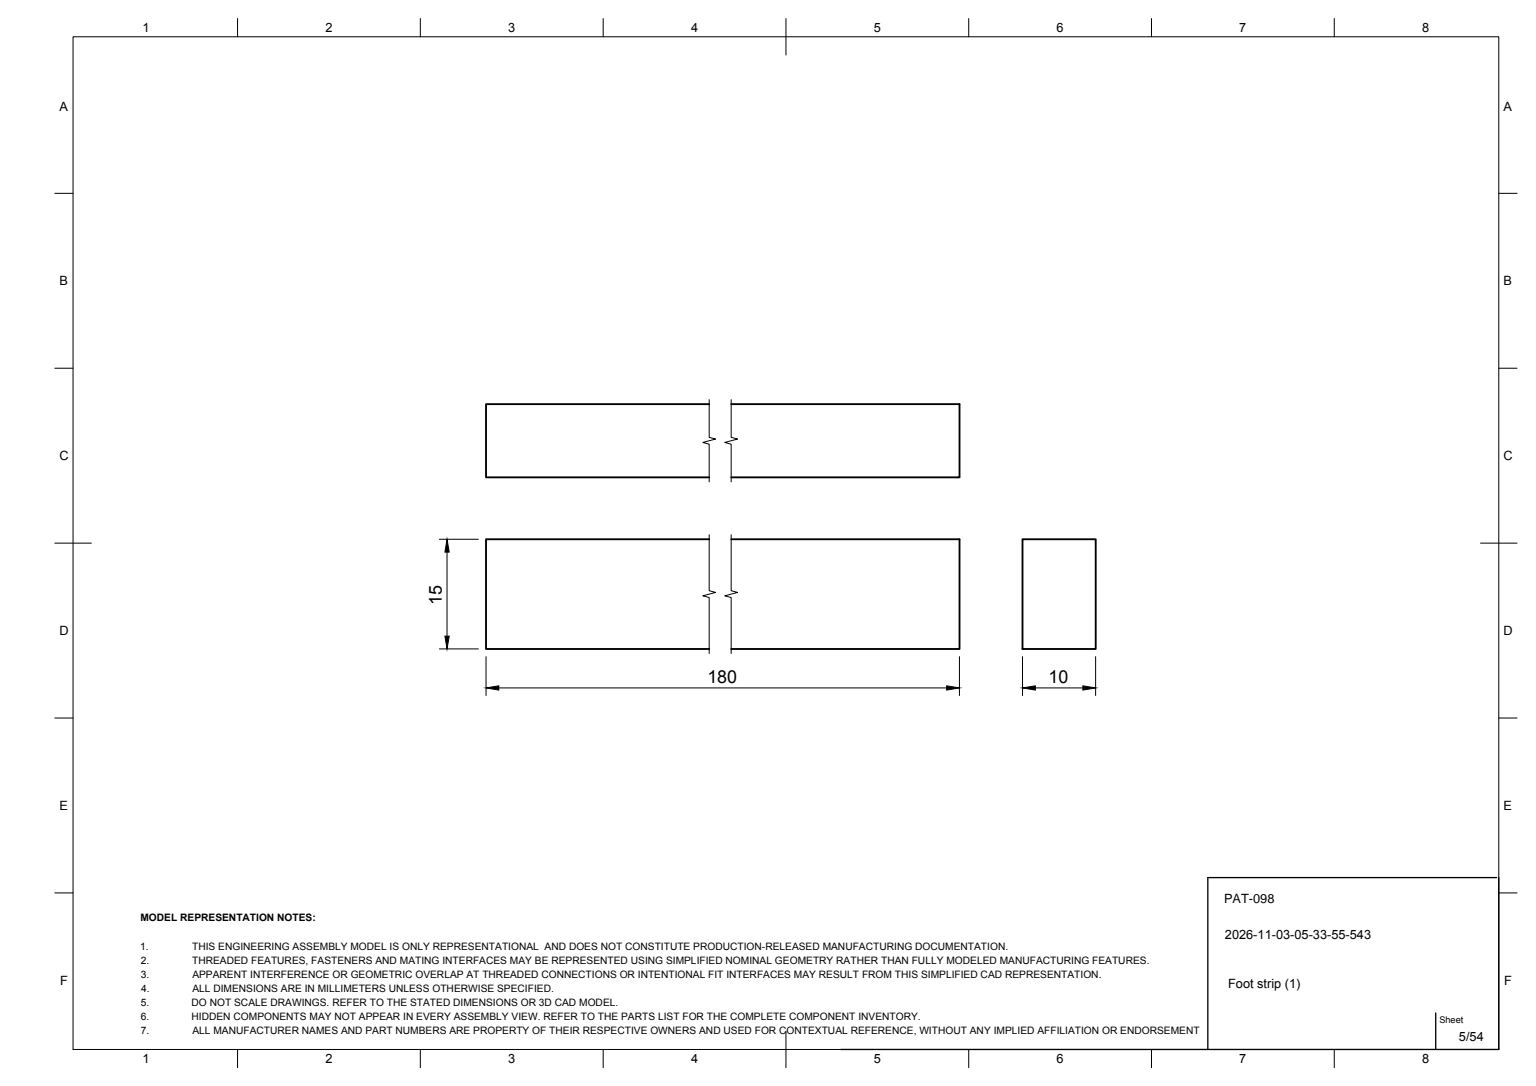
ISO-10303-21;
HEADER;
/* Generated by software containing ST-Developer
 * from STEP Tools, Inc. (www.steptools.com) 
 */

FILE_DESCRIPTION(
/* description */ ('Spring compression tester'),
/* implementation_level */ '2;1');

FILE_NAME(
/* name */ 'Foot strip (1).step',
/* time_stamp */ '2026-10-28T03:24:11-07:00',
/* author */ (''),
/* organization */ (''),
/* preprocessor_version */ 'ST-DEVELOPER v20.2',
/* originating_system */ 'Autodesk Translation Framework v15.17.0.0',
/* authorisation */ '');

FILE_SCHEMA (('AUTOMOTIVE_DESIGN { 1 0 10303 214 3 1 1 }'));
ENDSEC;

DATA;
#10=MECHANICAL_DESIGN_GEOMETRIC_PRESENTATION_REPRESENTATION('',(#1106),#43521);
#986=SHAPE_REPRESENTATION_RELATIONSHIP('SRR','None',#43798,#1046);
#1046=ADVANCED_BREP_SHAPE_REPRESENTATION('',(#1181),#43458);
#1106=STYLED_ITEM('',(#44188),#1181);
#1181=MANIFOLD_SOLID_BREP('Body1',#18543);
#1609=PLANE('',#19369);
#1610=PLANE('',#19370);
#1611=PLANE('',#19371);
#1612=PLANE('',#19372);
#1613=PLANE('',#19373);
#1614=PLANE('',#19374);
#2210=FACE_OUTER_BOUND('',#3293,.T.);
#2211=FACE_OUTER_BOUND('',#3294,.T.);
#2212=FACE_OUTER_BOUND('',#3295,.T.);
#2213=FACE_OUTER_BOUND('',#3296,.T.);
#2214=FACE_OUTER_BOUND('',#3297,.T.);
#2215=FACE_OUTER_BOUND('',#3298,.T.);
#3293=EDGE_LOOP('',(#12409,#12410,#12411,#12412));
#3294=EDGE_LOOP('',(#12413,#12414,#12415,#12416));
#3295=EDGE_LOOP('',(#12417,#12418,#12419,#12420));
#3296=EDGE_LOOP('',(#12421,#12422,#12423,#12424));
#3297=EDGE_LOOP('',(#12425,#12426,#12427,#12428));
#3298=EDGE_LOOP('',(#12429,#12430,#12431,#12432));
#4662=LINE('',#26660,#6094);
#4663=LINE('',#26662,#6095);
#4664=LINE('',#26664,#6096);
#4665=LINE('',#26665,#6097);
#4666=LINE('',#26668,#6098);
#4667=LINE('',#26670,#6099);
#4668=LINE('',#26671,#6100);
#4669=LINE('',#26674,#6101);
#4670=LINE('',#26676,#6102);
#4671=LINE('',#26677,#6103);
#4672=LINE('',#26679,#6104);
#4673=LINE('',#26680,#6105);
#6094=VECTOR('',#21424,1.);
#6095=VECTOR('',#21425,1.);
#6096=VECTOR('',#21426,1.);
#6097=VECTOR('',#21427,1.);
#6098=VECTOR('',#21430,1.);
#6099=VECTOR('',#21431,1.);
#6100=VECTOR('',#21432,1.);
#6101=VECTOR('',#21435,1.);
#6102=VECTOR('',#21436,1.);
#6103=VECTOR('',#21437,1.);
#6104=VECTOR('',#21440,1.);
#6105=VECTOR('',#21441,1.);
#8200=VERTEX_POINT('',#26658);
#8201=VERTEX_POINT('',#26659);
#8202=VERTEX_POINT('',#26661);
#8203=VERTEX_POINT('',#26663);
#8204=VERTEX_POINT('',#26667);
#8205=VERTEX_POINT('',#26669);
#8206=VERTEX_POINT('',#26673);
#8207=VERTEX_POINT('',#26675);
#9869=EDGE_CURVE('',#8200,#8201,#4662,.T.);
#9870=EDGE_CURVE('',#8201,#8202,#4663,.T.);
#9871=EDGE_CURVE('',#8203,#8202,#4664,.T.);
#9872=EDGE_CURVE('',#8200,#8203,#4665,.T.);
#9873=EDGE_CURVE('',#8204,#8200,#4666,.T.);
#9874=EDGE_CURVE('',#8205,#8203,#4667,.T.);
#9875=EDGE_CURVE('',#8204,#8205,#4668,.T.);
#9876=EDGE_CURVE('',#8206,#8204,#4669,.T.);
#9877=EDGE_CURVE('',#8207,#8205,#4670,.T.);
#9878=EDGE_CURVE('',#8206,#8207,#4671,.T.);
#9879=EDGE_CURVE('',#8201,#8206,#4672,.T.);
#9880=EDGE_CURVE('',#8202,#8207,#4673,.T.);
#12409=ORIENTED_EDGE('',*,*,#9869,.T.);
#12410=ORIENTED_EDGE('',*,*,#9870,.T.);
#12411=ORIENTED_EDGE('',*,*,#9871,.F.);
#12412=ORIENTED_EDGE('',*,*,#9872,.F.);
#12413=ORIENTED_EDGE('',*,*,#9873,.T.);
#12414=ORIENTED_EDGE('',*,*,#9872,.T.);
#12415=ORIENTED_EDGE('',*,*,#9874,.F.);
#12416=ORIENTED_EDGE('',*,*,#9875,.F.);
#12417=ORIENTED_EDGE('',*,*,#9876,.T.);
#12418=ORIENTED_EDGE('',*,*,#9875,.T.);
#12419=ORIENTED_EDGE('',*,*,#9877,.F.);
#12420=ORIENTED_EDGE('',*,*,#9878,.F.);
#12421=ORIENTED_EDGE('',*,*,#9879,.T.);
#12422=ORIENTED_EDGE('',*,*,#9878,.T.);
#12423=ORIENTED_EDGE('',*,*,#9880,.F.);
#12424=ORIENTED_EDGE('',*,*,#9870,.F.);
#12425=ORIENTED_EDGE('',*,*,#9880,.T.);
#12426=ORIENTED_EDGE('',*,*,#9877,.T.);
#12427=ORIENTED_EDGE('',*,*,#9874,.T.);
#12428=ORIENTED_EDGE('',*,*,#9871,.T.);
#12429=ORIENTED_EDGE('',*,*,#9879,.F.);
#12430=ORIENTED_EDGE('',*,*,#9869,.F.);
#12431=ORIENTED_EDGE('',*,*,#9873,.F.);
#12432=ORIENTED_EDGE('',*,*,#9876,.F.);
#17534=ADVANCED_FACE('',(#2210),#1609,.T.);
#17535=ADVANCED_FACE('',(#2211),#1610,.T.);
#17536=ADVANCED_FACE('',(#2212),#1611,.T.);
#17537=ADVANCED_FACE('',(#2213),#1612,.T.);
#17538=ADVANCED_FACE('',(#2214),#1613,.T.);
#17539=ADVANCED_FACE('',(#2215),#1614,.F.);
#18543=CLOSED_SHELL('',(#17534,#17535,#17536,#17537,#17538,#17539));
#19368=AXIS2_PLACEMENT_3D('',#26656,#21420,#21421);
#19369=AXIS2_PLACEMENT_3D('',#26657,#21422,#21423);
#19370=AXIS2_PLACEMENT_3D('',#26666,#21428,#21429);
#19371=AXIS2_PLACEMENT_3D('',#26672,#21433,#21434);
#19372=AXIS2_PLACEMENT_3D('',#26678,#21438,#21439);
#19373=AXIS2_PLACEMENT_3D('',#26681,#21442,#21443);
#19374=AXIS2_PLACEMENT_3D('',#26682,#21444,#21445);
#21420=DIRECTION('axis',(0.,0.,1.));
#21421=DIRECTION('refdir',(1.,0.,0.));
#21422=DIRECTION('center_axis',(0.,1.,0.));
#21423=DIRECTION('ref_axis',(-1.,0.,0.));
#21424=DIRECTION('',(-1.,0.,0.));
#21425=DIRECTION('',(0.,0.,1.));
#21426=DIRECTION('',(-1.,0.,0.));
#21427=DIRECTION('',(0.,0.,1.));
#21428=DIRECTION('center_axis',(1.,0.,0.));
#21429=DIRECTION('ref_axis',(0.,1.,0.));
#21430=DIRECTION('',(0.,1.,0.));
#21431=DIRECTION('',(0.,1.,0.));
#21432=DIRECTION('',(0.,0.,1.));
#21433=DIRECTION('center_axis',(0.,-1.,0.));
#21434=DIRECTION('ref_axis',(1.,0.,0.));
#21435=DIRECTION('',(1.,0.,0.));
#21436=DIRECTION('',(1.,0.,0.));
#21437=DIRECTION('',(0.,0.,1.));
#21438=DIRECTION('center_axis',(-1.,0.,0.));
#21439=DIRECTION('ref_axis',(0.,-1.,0.));
#21440=DIRECTION('',(0.,-1.,0.));
#21441=DIRECTION('',(0.,-1.,0.));
#21442=DIRECTION('center_axis',(0.,0.,1.));
#21443=DIRECTION('ref_axis',(1.,0.,0.));
#21444=DIRECTION('center_axis',(0.,0.,1.));
#21445=DIRECTION('ref_axis',(1.,0.,0.));
#26656=CARTESIAN_POINT('',(0.,0.,0.));
#26657=CARTESIAN_POINT('Origin',(9.,12.5,-2.2));
#26658=CARTESIAN_POINT('',(9.,12.5,-2.2));
#26659=CARTESIAN_POINT('',(-9.,12.5,-2.2));
#26660=CARTESIAN_POINT('',(9.,12.5,-2.2));
#26661=CARTESIAN_POINT('',(-9.,12.5,-1.2));
#26662=CARTESIAN_POINT('',(-9.,12.5,-2.2));
#26663=CARTESIAN_POINT('',(9.,12.5,-1.2));
#26664=CARTESIAN_POINT('',(9.,12.5,-1.2));
#26665=CARTESIAN_POINT('',(9.,12.5,-2.2));
#26666=CARTESIAN_POINT('Origin',(9.,11.,-2.2));
#26667=CARTESIAN_POINT('',(9.,11.,-2.2));
#26668=CARTESIAN_POINT('',(9.,11.,-2.2));
#26669=CARTESIAN_POINT('',(9.,11.,-1.2));
#26670=CARTESIAN_POINT('',(9.,11.,-1.2));
#26671=CARTESIAN_POINT('',(9.,11.,-2.2));
#26672=CARTESIAN_POINT('Origin',(-9.,11.,-2.2));
#26673=CARTESIAN_POINT('',(-9.,11.,-2.2));
#26674=CARTESIAN_POINT('',(-9.,11.,-2.2));
#26675=CARTESIAN_POINT('',(-9.,11.,-1.2));
#26676=CARTESIAN_POINT('',(-9.,11.,-1.2));
#26677=CARTESIAN_POINT('',(-9.,11.,-2.2));
#26678=CARTESIAN_POINT('Origin',(-9.,12.5,-2.2));
#26679=CARTESIAN_POINT('',(-9.,12.5,-2.2));
#26680=CARTESIAN_POINT('',(-9.,12.5,-1.2));
#26681=CARTESIAN_POINT('Origin',(0.,11.75,-1.2));
#26682=CARTESIAN_POINT('Origin',(0.,11.75,-2.2));
#43390=UNCERTAINTY_MEASURE_WITH_UNIT(LENGTH_MEASURE(0.001),#43522,
'DISTANCE_ACCURACY_VALUE',
'Maximum model space distance between geometric entities at asserted c
onnectivities');
#43453=UNCERTAINTY_MEASURE_WITH_UNIT(LENGTH_MEASURE(0.001),#43522,
'DISTANCE_ACCURACY_VALUE',
'Maximum model space distance between geometric entities at asserted c
onnectivities');
#43458=(
GEOMETRIC_REPRESENTATION_CONTEXT(3)
GLOBAL_UNCERTAINTY_ASSIGNED_CONTEXT((#43390))
GLOBAL_UNIT_ASSIGNED_CONTEXT((#43522,#43524,#43525))
REPRESENTATION_CONTEXT('','3D')
);
#43521=(
GEOMETRIC_REPRESENTATION_CONTEXT(3)
GLOBAL_UNCERTAINTY_ASSIGNED_CONTEXT((#43453))
GLOBAL_UNIT_ASSIGNED_CONTEXT((#43522,#43524,#43525))
REPRESENTATION_CONTEXT('','3D')
);
#43522=(
LENGTH_UNIT()
NAMED_UNIT(*)
SI_UNIT(.CENTI.,.METRE.)
);
#43524=(
NAMED_UNIT(*)
PLANE_ANGLE_UNIT()
SI_UNIT($,.RADIAN.)
);
#43525=(
NAMED_UNIT(*)
SI_UNIT($,.STERADIAN.)
SOLID_ANGLE_UNIT()
);
#43530=SHAPE_DEFINITION_REPRESENTATION(#43597,#43798);
#43597=PRODUCT_DEFINITION_SHAPE('',$,#43866);
#43798=SHAPE_REPRESENTATION('',(#19368),#43458);
#43861=PRODUCT_DEFINITION_CONTEXT('part definition',#44064,'design');
#43866=PRODUCT_DEFINITION('Foot strip (1)','Foot strip (1)',#43933,#43861);
#43933=PRODUCT_DEFINITION_FORMATION('',$,#44070);
#44064=APPLICATION_CONTEXT(
'Core Data for Automotive Mechanical Design Process');
#44065=PRODUCT_CONTEXT('part definition',#44064,'mechanical');
#44070=PRODUCT('Foot strip (1)','Foot strip (1)','Foot strip (1)',(#44065));
#44182=COLOUR_RGB('Light Blue',0.38,0.62,0.78);
#44183=FILL_AREA_STYLE_COLOUR('',#44182);
#44184=FILL_AREA_STYLE('',(#44183));
#44185=SURFACE_STYLE_FILL_AREA(#44184);
#44186=SURFACE_SIDE_STYLE('',(#44185));
#44187=SURFACE_STYLE_USAGE(.BOTH.,#44186);
#44188=PRESENTATION_STYLE_ASSIGNMENT((#44187));
ENDSEC;
END-ISO-10303-21;
